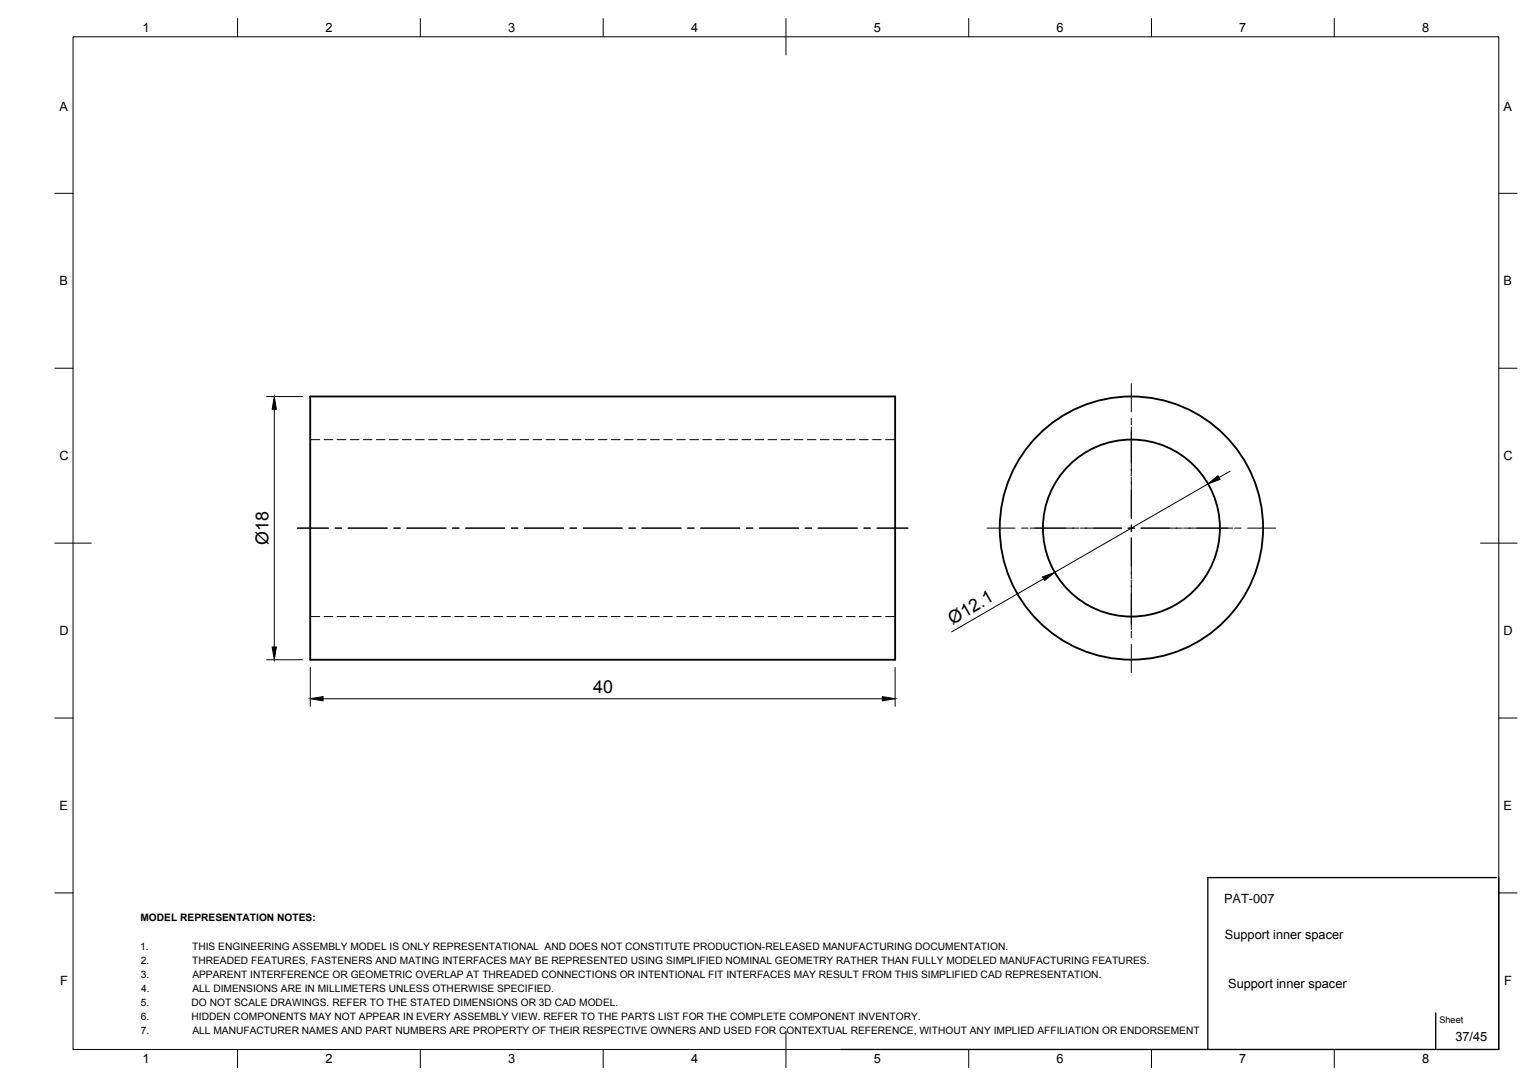
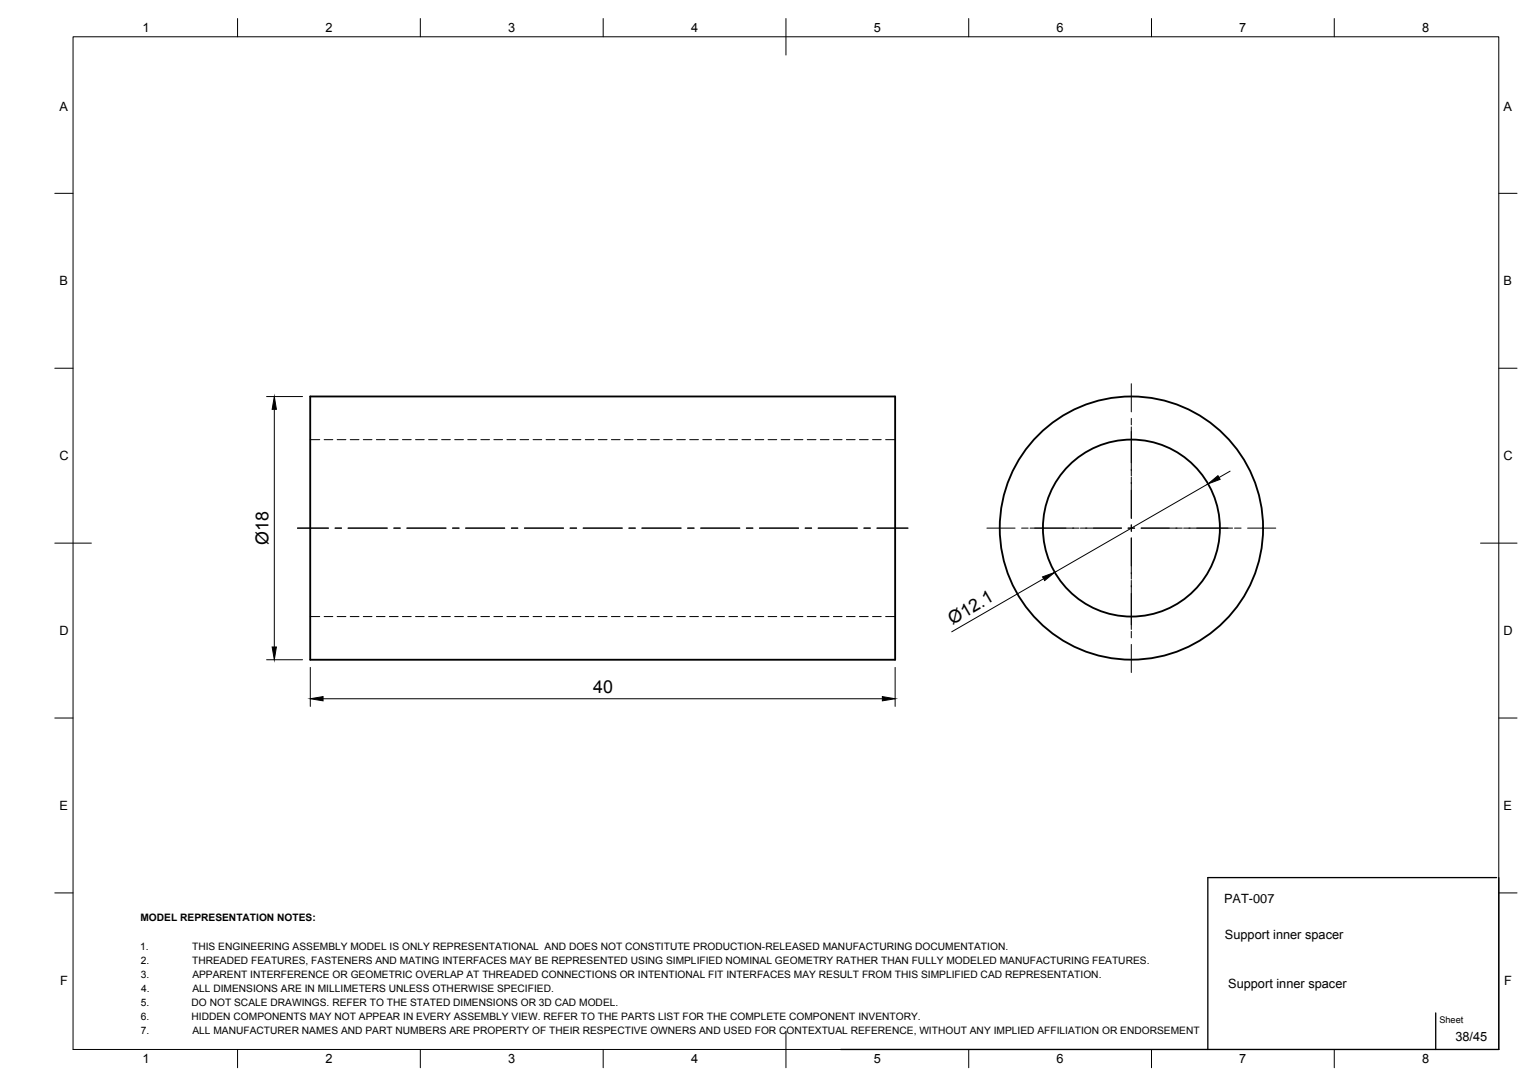
ISO-10303-21;
HEADER;
/* Generated by software containing ST-Developer
 * from STEP Tools, Inc. (www.steptools.com) 
 */

FILE_DESCRIPTION(
/* description */ ('Bearing friction torque test rig'),
/* implementation_level */ '2;1');

FILE_NAME(
/* name */ 'Support inner spacer.step',
/* time_stamp */ '2026-10-28T03:24:04-07:00',
/* author */ (''),
/* organization */ (''),
/* preprocessor_version */ 'ST-DEVELOPER v20.2',
/* originating_system */ 'Autodesk Translation Framework v15.17.0.0',
/* authorisation */ '');

FILE_SCHEMA (('AUTOMOTIVE_DESIGN { 1 0 10303 214 3 1 1 }'));
ENDSEC;

DATA;
#10=MECHANICAL_DESIGN_GEOMETRIC_PRESENTATION_REPRESENTATION('',(#583),#14822);
#490=SHAPE_REPRESENTATION_RELATIONSHIP('SRR','None',#15032,#529);
#529=ADVANCED_BREP_SHAPE_REPRESENTATION('',(#634),#14812);
#583=STYLED_ITEM('',(#15298),#634);
#634=MANIFOLD_SOLID_BREP('Body1',#7702);
#836=FACE_BOUND('',#2115,.T.);
#837=FACE_BOUND('',#2117,.T.);
#1061=PLANE('',#9012);
#1062=PLANE('',#9013);
#1475=FACE_OUTER_BOUND('',#2112,.T.);
#1476=FACE_OUTER_BOUND('',#2113,.T.);
#1477=FACE_OUTER_BOUND('',#2114,.T.);
#1478=FACE_OUTER_BOUND('',#2116,.T.);
#2112=EDGE_LOOP('',(#6756,#6757,#6758,#6759));
#2113=EDGE_LOOP('',(#6760,#6761,#6762,#6763));
#2114=EDGE_LOOP('',(#6764));
#2115=EDGE_LOOP('',(#6765));
#2116=EDGE_LOOP('',(#6766));
#2117=EDGE_LOOP('',(#6767));
#2604=LINE('',#14125,#3048);
#2605=LINE('',#14131,#3049);
#3048=VECTOR('',#11283,0.605);
#3049=VECTOR('',#11290,0.9);
#3488=CIRCLE('',#9007,0.605);
#3489=CIRCLE('',#9008,0.605);
#3490=CIRCLE('',#9010,0.9);
#3491=CIRCLE('',#9011,0.9);
#4103=VERTEX_POINT('',#14122);
#4104=VERTEX_POINT('',#14124);
#4105=VERTEX_POINT('',#14128);
#4106=VERTEX_POINT('',#14130);
#5004=EDGE_CURVE('',#4103,#4103,#3488,.T.);
#5005=EDGE_CURVE('',#4103,#4104,#2604,.T.);
#5006=EDGE_CURVE('',#4104,#4104,#3489,.T.);
#5007=EDGE_CURVE('',#4105,#4105,#3490,.T.);
#5008=EDGE_CURVE('',#4105,#4106,#2605,.T.);
#5009=EDGE_CURVE('',#4106,#4106,#3491,.T.);
#6756=ORIENTED_EDGE('',*,*,#5004,.F.);
#6757=ORIENTED_EDGE('',*,*,#5005,.T.);
#6758=ORIENTED_EDGE('',*,*,#5006,.T.);
#6759=ORIENTED_EDGE('',*,*,#5005,.F.);
#6760=ORIENTED_EDGE('',*,*,#5007,.F.);
#6761=ORIENTED_EDGE('',*,*,#5008,.T.);
#6762=ORIENTED_EDGE('',*,*,#5009,.T.);
#6763=ORIENTED_EDGE('',*,*,#5008,.F.);
#6764=ORIENTED_EDGE('',*,*,#5007,.T.);
#6765=ORIENTED_EDGE('',*,*,#5004,.T.);
#6766=ORIENTED_EDGE('',*,*,#5009,.F.);
#6767=ORIENTED_EDGE('',*,*,#5006,.F.);
#7181=CYLINDRICAL_SURFACE('',#9006,0.605);
#7182=CYLINDRICAL_SURFACE('',#9009,0.9);
#7586=ADVANCED_FACE('',(#1475),#7181,.F.);
#7587=ADVANCED_FACE('',(#1476),#7182,.T.);
#7588=ADVANCED_FACE('',(#1477,#836),#1061,.T.);
#7589=ADVANCED_FACE('',(#1478,#837),#1062,.F.);
#7702=CLOSED_SHELL('',(#7586,#7587,#7588,#7589));
#9005=AXIS2_PLACEMENT_3D('',#14120,#11277,#11278);
#9006=AXIS2_PLACEMENT_3D('',#14121,#11279,#11280);
#9007=AXIS2_PLACEMENT_3D('',#14123,#11281,#11282);
#9008=AXIS2_PLACEMENT_3D('',#14126,#11284,#11285);
#9009=AXIS2_PLACEMENT_3D('',#14127,#11286,#11287);
#9010=AXIS2_PLACEMENT_3D('',#14129,#11288,#11289);
#9011=AXIS2_PLACEMENT_3D('',#14132,#11291,#11292);
#9012=AXIS2_PLACEMENT_3D('',#14133,#11293,#11294);
#9013=AXIS2_PLACEMENT_3D('',#14134,#11295,#11296);
#11277=DIRECTION('axis',(0.,0.,1.));
#11278=DIRECTION('refdir',(1.,0.,0.));
#11279=DIRECTION('center_axis',(0.,1.,0.));
#11280=DIRECTION('ref_axis',(1.,0.,0.));
#11281=DIRECTION('center_axis',(0.,-1.,0.));
#11282=DIRECTION('ref_axis',(1.,0.,0.));
#11283=DIRECTION('',(0.,-1.,0.));
#11284=DIRECTION('center_axis',(0.,-1.,0.));
#11285=DIRECTION('ref_axis',(1.,0.,0.));
#11286=DIRECTION('center_axis',(0.,1.,0.));
#11287=DIRECTION('ref_axis',(1.,0.,0.));
#11288=DIRECTION('center_axis',(0.,1.,0.));
#11289=DIRECTION('ref_axis',(1.,0.,0.));
#11290=DIRECTION('',(0.,-1.,0.));
#11291=DIRECTION('center_axis',(0.,1.,0.));
#11292=DIRECTION('ref_axis',(1.,0.,0.));
#11293=DIRECTION('center_axis',(0.,1.,0.));
#11294=DIRECTION('ref_axis',(1.,0.,0.));
#11295=DIRECTION('center_axis',(0.,1.,0.));
#11296=DIRECTION('ref_axis',(1.,0.,0.));
#14120=CARTESIAN_POINT('',(0.,0.,0.));
#14121=CARTESIAN_POINT('Origin',(0.,-6.5,7.));
#14122=CARTESIAN_POINT('',(-0.605,-2.5,7.));
#14123=CARTESIAN_POINT('Origin',(0.,-2.5,7.));
#14124=CARTESIAN_POINT('',(-0.605,-6.5,7.));
#14125=CARTESIAN_POINT('',(-0.605,-6.5,7.));
#14126=CARTESIAN_POINT('Origin',(0.,-6.5,7.));
#14127=CARTESIAN_POINT('Origin',(0.,-6.5,7.));
#14128=CARTESIAN_POINT('',(-0.9,-2.5,7.));
#14129=CARTESIAN_POINT('Origin',(0.,-2.5,7.));
#14130=CARTESIAN_POINT('',(-0.9,-6.5,7.));
#14131=CARTESIAN_POINT('',(-0.9,-6.5,7.));
#14132=CARTESIAN_POINT('Origin',(0.,-6.5,7.));
#14133=CARTESIAN_POINT('Origin',(0.,-2.5,7.));
#14134=CARTESIAN_POINT('Origin',(0.,-6.5,7.));
#14767=UNCERTAINTY_MEASURE_WITH_UNIT(LENGTH_MEASURE(0.001),#14823,
'DISTANCE_ACCURACY_VALUE',
'Maximum model space distance between geometric entities at asserted c
onnectivities');
#14777=UNCERTAINTY_MEASURE_WITH_UNIT(LENGTH_MEASURE(0.001),#14823,
'DISTANCE_ACCURACY_VALUE',
'Maximum model space distance between geometric entities at asserted c
onnectivities');
#14812=(
GEOMETRIC_REPRESENTATION_CONTEXT(3)
GLOBAL_UNCERTAINTY_ASSIGNED_CONTEXT((#14767))
GLOBAL_UNIT_ASSIGNED_CONTEXT((#14823,#14825,#14826))
REPRESENTATION_CONTEXT('','3D')
);
#14822=(
GEOMETRIC_REPRESENTATION_CONTEXT(3)
GLOBAL_UNCERTAINTY_ASSIGNED_CONTEXT((#14777))
GLOBAL_UNIT_ASSIGNED_CONTEXT((#14823,#14825,#14826))
REPRESENTATION_CONTEXT('','3D')
);
#14823=(
LENGTH_UNIT()
NAMED_UNIT(*)
SI_UNIT(.CENTI.,.METRE.)
);
#14825=(
NAMED_UNIT(*)
PLANE_ANGLE_UNIT()
SI_UNIT($,.RADIAN.)
);
#14826=(
NAMED_UNIT(*)
SI_UNIT($,.STERADIAN.)
SOLID_ANGLE_UNIT()
);
#14861=SHAPE_DEFINITION_REPRESENTATION(#14971,#15032);
#14971=PRODUCT_DEFINITION_SHAPE('',$,#15077);
#15032=SHAPE_REPRESENTATION('',(#9005),#14812);
#15042=PRODUCT_DEFINITION_CONTEXT('part definition',#15176,'design');
#15077=PRODUCT_DEFINITION('Support inner spacer','Support inner spacer',
#15121,#15042);
#15121=PRODUCT_DEFINITION_FORMATION('',$,#15212);
#15176=APPLICATION_CONTEXT(
'Core Data for Automotive Mechanical Design Process');
#15177=PRODUCT_CONTEXT('part definition',#15176,'mechanical');
#15212=PRODUCT('Support inner spacer','Support inner spacer',
'Support inner spacer',(#15177));
#15292=COLOUR_RGB('Off White',0.89,0.88,0.83);
#15293=FILL_AREA_STYLE_COLOUR('',#15292);
#15294=FILL_AREA_STYLE('',(#15293));
#15295=SURFACE_STYLE_FILL_AREA(#15294);
#15296=SURFACE_SIDE_STYLE('',(#15295));
#15297=SURFACE_STYLE_USAGE(.BOTH.,#15296);
#15298=PRESENTATION_STYLE_ASSIGNMENT((#15297));
ENDSEC;
END-ISO-10303-21;
